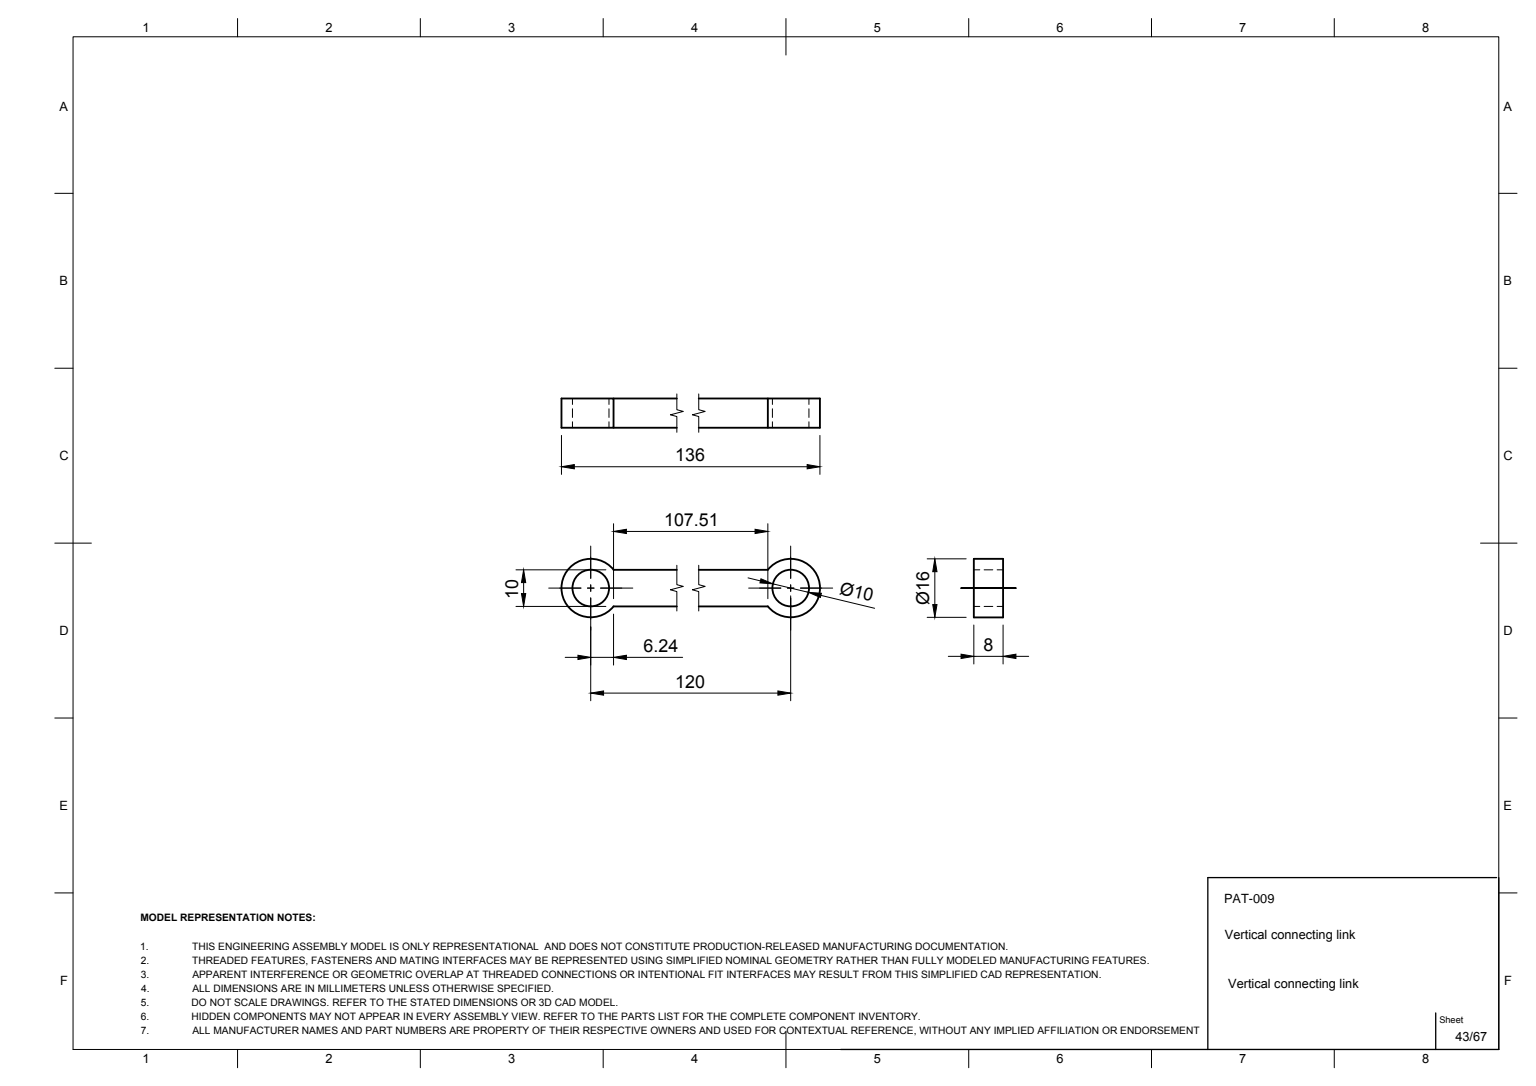
ISO-10303-21;
HEADER;
/* Generated by software containing ST-Developer
 * from STEP Tools, Inc. (www.steptools.com) 
 */

FILE_DESCRIPTION(
/* description */ ('Bell-crank linkage with push rods'),
/* implementation_level */ '2;1');

FILE_NAME(
/* name */ 'Vertical connecting link.step',
/* time_stamp */ '2026-10-28T03:25:15-07:00',
/* author */ (''),
/* organization */ (''),
/* preprocessor_version */ 'ST-DEVELOPER v20.2',
/* originating_system */ 'Autodesk Translation Framework v15.17.0.0',
/* authorisation */ '');

FILE_SCHEMA (('AUTOMOTIVE_DESIGN { 1 0 10303 214 3 1 1 }'));
ENDSEC;

DATA;
#10=MECHANICAL_DESIGN_GEOMETRIC_PRESENTATION_REPRESENTATION('',(#646),#16678);
#530=SHAPE_REPRESENTATION_RELATIONSHIP('SRR','None',#16950,#584);
#584=ADVANCED_BREP_SHAPE_REPRESENTATION('',(#706),#16655);
#646=STYLED_ITEM('',(#17277),#706);
#706=MANIFOLD_SOLID_BREP('Body1',#8838);
#866=FACE_BOUND('',#2268,.T.);
#867=FACE_BOUND('',#2269,.T.);
#868=FACE_BOUND('',#2273,.T.);
#869=FACE_BOUND('',#2274,.T.);
#1151=PLANE('',#10206);
#1152=PLANE('',#10207);
#1153=PLANE('',#10209);
#1154=PLANE('',#10212);
#1600=FACE_OUTER_BOUND('',#2263,.T.);
#1601=FACE_OUTER_BOUND('',#2264,.T.);
#1602=FACE_OUTER_BOUND('',#2265,.T.);
#1603=FACE_OUTER_BOUND('',#2266,.T.);
#1604=FACE_OUTER_BOUND('',#2267,.T.);
#1605=FACE_OUTER_BOUND('',#2270,.T.);
#1606=FACE_OUTER_BOUND('',#2271,.T.);
#1607=FACE_OUTER_BOUND('',#2272,.T.);
#2263=EDGE_LOOP('',(#7395,#7396,#7397,#7398));
#2264=EDGE_LOOP('',(#7399,#7400,#7401,#7402));
#2265=EDGE_LOOP('',(#7403,#7404,#7405,#7406));
#2266=EDGE_LOOP('',(#7407,#7408,#7409,#7410));
#2267=EDGE_LOOP('',(#7411,#7412,#7413,#7414));
#2268=EDGE_LOOP('',(#7415));
#2269=EDGE_LOOP('',(#7416));
#2270=EDGE_LOOP('',(#7417,#7418,#7419,#7420));
#2271=EDGE_LOOP('',(#7421,#7422,#7423,#7424));
#2272=EDGE_LOOP('',(#7425,#7426,#7427,#7428));
#2273=EDGE_LOOP('',(#7429));
#2274=EDGE_LOOP('',(#7430));
#2894=LINE('',#15712,#3443);
#2895=LINE('',#15718,#3444);
#2896=LINE('',#15723,#3445);
#2897=LINE('',#15727,#3446);
#2898=LINE('',#15731,#3447);
#2899=LINE('',#15733,#3448);
#2900=LINE('',#15734,#3449);
#2901=LINE('',#15737,#3450);
#2902=LINE('',#15741,#3451);
#2903=LINE('',#15742,#3452);
#3443=VECTOR('',#12482,0.5);
#3444=VECTOR('',#12489,0.5);
#3445=VECTOR('',#12494,1.);
#3446=VECTOR('',#12497,1.);
#3447=VECTOR('',#12502,1.);
#3448=VECTOR('',#12503,1.);
#3449=VECTOR('',#12504,1.);
#3450=VECTOR('',#12507,1.);
#3451=VECTOR('',#12512,1.);
#3452=VECTOR('',#12513,1.);
#3971=CIRCLE('',#10198,0.5);
#3972=CIRCLE('',#10199,0.5);
#3973=CIRCLE('',#10201,0.5);
#3974=CIRCLE('',#10202,0.5);
#3975=CIRCLE('',#10204,0.8);
#3976=CIRCLE('',#10205,0.8);
#3977=CIRCLE('',#10208,0.8);
#3978=CIRCLE('',#10211,0.8);
#4610=VERTEX_POINT('',#15709);
#4611=VERTEX_POINT('',#15711);
#4612=VERTEX_POINT('',#15715);
#4613=VERTEX_POINT('',#15717);
#4614=VERTEX_POINT('',#15721);
#4615=VERTEX_POINT('',#15722);
#4616=VERTEX_POINT('',#15724);
#4617=VERTEX_POINT('',#15726);
#4618=VERTEX_POINT('',#15730);
#4619=VERTEX_POINT('',#15732);
#4620=VERTEX_POINT('',#15736);
#4621=VERTEX_POINT('',#15740);
#5575=EDGE_CURVE('',#4610,#4610,#3971,.T.);
#5576=EDGE_CURVE('',#4610,#4611,#2894,.T.);
#5577=EDGE_CURVE('',#4611,#4611,#3972,.T.);
#5578=EDGE_CURVE('',#4612,#4612,#3973,.T.);
#5579=EDGE_CURVE('',#4612,#4613,#2895,.T.);
#5580=EDGE_CURVE('',#4613,#4613,#3974,.T.);
#5581=EDGE_CURVE('',#4614,#4615,#2896,.T.);
#5582=EDGE_CURVE('',#4616,#4614,#3975,.T.);
#5583=EDGE_CURVE('',#4617,#4616,#2897,.T.);
#5584=EDGE_CURVE('',#4617,#4615,#3976,.T.);
#5585=EDGE_CURVE('',#4618,#4615,#2898,.T.);
#5586=EDGE_CURVE('',#4619,#4618,#2899,.T.);
#5587=EDGE_CURVE('',#4614,#4619,#2900,.T.);
#5588=EDGE_CURVE('',#4617,#4620,#2901,.T.);
#5589=EDGE_CURVE('',#4618,#4620,#3977,.T.);
#5590=EDGE_CURVE('',#4621,#4616,#2902,.T.);
#5591=EDGE_CURVE('',#4620,#4621,#2903,.T.);
#5592=EDGE_CURVE('',#4619,#4621,#3978,.T.);
#7395=ORIENTED_EDGE('',*,*,#5575,.F.);
#7396=ORIENTED_EDGE('',*,*,#5576,.T.);
#7397=ORIENTED_EDGE('',*,*,#5577,.F.);
#7398=ORIENTED_EDGE('',*,*,#5576,.F.);
#7399=ORIENTED_EDGE('',*,*,#5578,.F.);
#7400=ORIENTED_EDGE('',*,*,#5579,.T.);
#7401=ORIENTED_EDGE('',*,*,#5580,.F.);
#7402=ORIENTED_EDGE('',*,*,#5579,.F.);
#7403=ORIENTED_EDGE('',*,*,#5581,.F.);
#7404=ORIENTED_EDGE('',*,*,#5582,.F.);
#7405=ORIENTED_EDGE('',*,*,#5583,.F.);
#7406=ORIENTED_EDGE('',*,*,#5584,.T.);
#7407=ORIENTED_EDGE('',*,*,#5581,.T.);
#7408=ORIENTED_EDGE('',*,*,#5585,.F.);
#7409=ORIENTED_EDGE('',*,*,#5586,.F.);
#7410=ORIENTED_EDGE('',*,*,#5587,.F.);
#7411=ORIENTED_EDGE('',*,*,#5584,.F.);
#7412=ORIENTED_EDGE('',*,*,#5588,.T.);
#7413=ORIENTED_EDGE('',*,*,#5589,.F.);
#7414=ORIENTED_EDGE('',*,*,#5585,.T.);
#7415=ORIENTED_EDGE('',*,*,#5575,.T.);
#7416=ORIENTED_EDGE('',*,*,#5578,.T.);
#7417=ORIENTED_EDGE('',*,*,#5583,.T.);
#7418=ORIENTED_EDGE('',*,*,#5590,.F.);
#7419=ORIENTED_EDGE('',*,*,#5591,.F.);
#7420=ORIENTED_EDGE('',*,*,#5588,.F.);
#7421=ORIENTED_EDGE('',*,*,#5586,.T.);
#7422=ORIENTED_EDGE('',*,*,#5589,.T.);
#7423=ORIENTED_EDGE('',*,*,#5591,.T.);
#7424=ORIENTED_EDGE('',*,*,#5592,.F.);
#7425=ORIENTED_EDGE('',*,*,#5587,.T.);
#7426=ORIENTED_EDGE('',*,*,#5592,.T.);
#7427=ORIENTED_EDGE('',*,*,#5590,.T.);
#7428=ORIENTED_EDGE('',*,*,#5582,.T.);
#7429=ORIENTED_EDGE('',*,*,#5577,.T.);
#7430=ORIENTED_EDGE('',*,*,#5580,.T.);
#8202=CYLINDRICAL_SURFACE('',#10197,0.5);
#8203=CYLINDRICAL_SURFACE('',#10200,0.5);
#8204=CYLINDRICAL_SURFACE('',#10203,0.8);
#8205=CYLINDRICAL_SURFACE('',#10210,0.8);
#8625=ADVANCED_FACE('',(#1600),#8202,.F.);
#8626=ADVANCED_FACE('',(#1601),#8203,.F.);
#8627=ADVANCED_FACE('',(#1602),#8204,.T.);
#8628=ADVANCED_FACE('',(#1603),#1151,.T.);
#8629=ADVANCED_FACE('',(#1604,#866,#867),#1152,.F.);
#8630=ADVANCED_FACE('',(#1605),#1153,.T.);
#8631=ADVANCED_FACE('',(#1606),#8205,.T.);
#8632=ADVANCED_FACE('',(#1607,#868,#869),#1154,.T.);
#8838=CLOSED_SHELL('',(#8625,#8626,#8627,#8628,#8629,#8630,#8631,#8632));
#10196=AXIS2_PLACEMENT_3D('',#15707,#12476,#12477);
#10197=AXIS2_PLACEMENT_3D('',#15708,#12478,#12479);
#10198=AXIS2_PLACEMENT_3D('',#15710,#12480,#12481);
#10199=AXIS2_PLACEMENT_3D('',#15713,#12483,#12484);
#10200=AXIS2_PLACEMENT_3D('',#15714,#12485,#12486);
#10201=AXIS2_PLACEMENT_3D('',#15716,#12487,#12488);
#10202=AXIS2_PLACEMENT_3D('',#15719,#12490,#12491);
#10203=AXIS2_PLACEMENT_3D('',#15720,#12492,#12493);
#10204=AXIS2_PLACEMENT_3D('',#15725,#12495,#12496);
#10205=AXIS2_PLACEMENT_3D('',#15728,#12498,#12499);
#10206=AXIS2_PLACEMENT_3D('',#15729,#12500,#12501);
#10207=AXIS2_PLACEMENT_3D('',#15735,#12505,#12506);
#10208=AXIS2_PLACEMENT_3D('',#15738,#12508,#12509);
#10209=AXIS2_PLACEMENT_3D('',#15739,#12510,#12511);
#10210=AXIS2_PLACEMENT_3D('',#15743,#12514,#12515);
#10211=AXIS2_PLACEMENT_3D('',#15744,#12516,#12517);
#10212=AXIS2_PLACEMENT_3D('',#15745,#12518,#12519);
#12476=DIRECTION('axis',(0.,0.,1.));
#12477=DIRECTION('refdir',(1.,0.,0.));
#12478=DIRECTION('center_axis',(0.,0.,1.));
#12479=DIRECTION('ref_axis',(1.,0.,0.));
#12480=DIRECTION('center_axis',(0.,0.,1.));
#12481=DIRECTION('ref_axis',(1.,0.,0.));
#12482=DIRECTION('',(0.,0.,1.));
#12483=DIRECTION('center_axis',(0.,0.,-1.));
#12484=DIRECTION('ref_axis',(1.,0.,0.));
#12485=DIRECTION('center_axis',(0.,0.,1.));
#12486=DIRECTION('ref_axis',(1.,0.,0.));
#12487=DIRECTION('center_axis',(0.,0.,1.));
#12488=DIRECTION('ref_axis',(1.,0.,0.));
#12489=DIRECTION('',(0.,0.,1.));
#12490=DIRECTION('center_axis',(0.,0.,-1.));
#12491=DIRECTION('ref_axis',(1.,0.,0.));
#12492=DIRECTION('center_axis',(0.,0.,1.));
#12493=DIRECTION('ref_axis',(-1.83697019872103E-16,1.,0.));
#12494=DIRECTION('',(0.,0.,-1.));
#12495=DIRECTION('center_axis',(0.,0.,1.));
#12496=DIRECTION('ref_axis',(1.,0.,0.));
#12497=DIRECTION('',(0.,0.,1.));
#12498=DIRECTION('center_axis',(0.,0.,1.));
#12499=DIRECTION('ref_axis',(1.,0.,0.));
#12500=DIRECTION('center_axis',(-1.,0.,0.));
#12501=DIRECTION('ref_axis',(0.,-1.,0.));
#12502=DIRECTION('',(0.,1.,0.));
#12503=DIRECTION('',(0.,0.,-1.));
#12504=DIRECTION('',(0.,-1.,0.));
#12505=DIRECTION('center_axis',(0.,0.,1.));
#12506=DIRECTION('ref_axis',(1.,0.,0.));
#12507=DIRECTION('',(0.,-1.,0.));
#12508=DIRECTION('center_axis',(0.,0.,1.));
#12509=DIRECTION('ref_axis',(1.,0.,0.));
#12510=DIRECTION('center_axis',(1.,0.,0.));
#12511=DIRECTION('ref_axis',(0.,1.,0.));
#12512=DIRECTION('',(0.,1.,0.));
#12513=DIRECTION('',(0.,0.,1.));
#12514=DIRECTION('center_axis',(0.,0.,1.));
#12515=DIRECTION('ref_axis',(-1.83697019872103E-16,-1.,0.));
#12516=DIRECTION('center_axis',(0.,0.,1.));
#12517=DIRECTION('ref_axis',(1.,0.,0.));
#12518=DIRECTION('center_axis',(0.,0.,1.));
#12519=DIRECTION('ref_axis',(1.,0.,0.));
#15707=CARTESIAN_POINT('',(0.,0.,0.));
#15708=CARTESIAN_POINT('Origin',(4.,0.,6.7));
#15709=CARTESIAN_POINT('',(3.5,-6.12323399573677E-17,6.8));
#15710=CARTESIAN_POINT('Origin',(4.,0.,6.8));
#15711=CARTESIAN_POINT('',(3.5,6.12323399573677E-17,7.6));
#15712=CARTESIAN_POINT('',(3.5,-6.12323399573677E-17,6.7));
#15713=CARTESIAN_POINT('Origin',(4.,0.,7.6));
#15714=CARTESIAN_POINT('Origin',(4.,12.,6.7));
#15715=CARTESIAN_POINT('',(3.5,12.,6.8));
#15716=CARTESIAN_POINT('Origin',(4.,12.,6.8));
#15717=CARTESIAN_POINT('',(3.5,12.,7.6));
#15718=CARTESIAN_POINT('',(3.5,12.,6.7));
#15719=CARTESIAN_POINT('Origin',(4.,12.,7.6));
#15720=CARTESIAN_POINT('Origin',(4.,12.,6.8));
#15721=CARTESIAN_POINT('',(3.5,11.3755002001602,7.6));
#15722=CARTESIAN_POINT('',(3.5,11.3755002001602,6.8));
#15723=CARTESIAN_POINT('',(3.5,11.3755002001602,6.8));
#15724=CARTESIAN_POINT('',(4.5,11.3755002001602,7.6));
#15725=CARTESIAN_POINT('Origin',(4.,12.,7.6));
#15726=CARTESIAN_POINT('',(4.5,11.3755002001602,6.8));
#15727=CARTESIAN_POINT('',(4.5,11.3755002001602,6.8));
#15728=CARTESIAN_POINT('Origin',(4.,12.,6.8));
#15729=CARTESIAN_POINT('Origin',(3.5,12.,6.8));
#15730=CARTESIAN_POINT('',(3.5,0.62449979983984,6.8));
#15731=CARTESIAN_POINT('',(3.5,0.,6.8));
#15732=CARTESIAN_POINT('',(3.5,0.62449979983984,7.6));
#15733=CARTESIAN_POINT('',(3.5,0.62449979983984,6.8));
#15734=CARTESIAN_POINT('',(3.5,0.,7.6));
#15735=CARTESIAN_POINT('Origin',(4.,0.,6.8));
#15736=CARTESIAN_POINT('',(4.5,0.62449979983984,6.8));
#15737=CARTESIAN_POINT('',(4.5,12.,6.8));
#15738=CARTESIAN_POINT('Origin',(4.,0.,6.8));
#15739=CARTESIAN_POINT('Origin',(4.5,0.,6.8));
#15740=CARTESIAN_POINT('',(4.5,0.62449979983984,7.6));
#15741=CARTESIAN_POINT('',(4.5,12.,7.6));
#15742=CARTESIAN_POINT('',(4.5,0.62449979983984,6.8));
#15743=CARTESIAN_POINT('Origin',(4.,0.,6.8));
#15744=CARTESIAN_POINT('Origin',(4.,0.,7.6));
#15745=CARTESIAN_POINT('Origin',(4.,0.,7.6));
#16591=UNCERTAINTY_MEASURE_WITH_UNIT(LENGTH_MEASURE(0.001),#16679,
'DISTANCE_ACCURACY_VALUE',
'Maximum model space distance between geometric entities at asserted c
onnectivities');
#16614=UNCERTAINTY_MEASURE_WITH_UNIT(LENGTH_MEASURE(0.001),#16679,
'DISTANCE_ACCURACY_VALUE',
'Maximum model space distance between geometric entities at asserted c
onnectivities');
#16655=(
GEOMETRIC_REPRESENTATION_CONTEXT(3)
GLOBAL_UNCERTAINTY_ASSIGNED_CONTEXT((#16591))
GLOBAL_UNIT_ASSIGNED_CONTEXT((#16679,#16681,#16682))
REPRESENTATION_CONTEXT('','3D')
);
#16678=(
GEOMETRIC_REPRESENTATION_CONTEXT(3)
GLOBAL_UNCERTAINTY_ASSIGNED_CONTEXT((#16614))
GLOBAL_UNIT_ASSIGNED_CONTEXT((#16679,#16681,#16682))
REPRESENTATION_CONTEXT('','3D')
);
#16679=(
LENGTH_UNIT()
NAMED_UNIT(*)
SI_UNIT(.CENTI.,.METRE.)
);
#16681=(
NAMED_UNIT(*)
PLANE_ANGLE_UNIT()
SI_UNIT($,.RADIAN.)
);
#16682=(
NAMED_UNIT(*)
SI_UNIT($,.STERADIAN.)
SOLID_ANGLE_UNIT()
);
#16723=SHAPE_DEFINITION_REPRESENTATION(#16794,#16950);
#16794=PRODUCT_DEFINITION_SHAPE('',$,#17014);
#16950=SHAPE_REPRESENTATION('',(#10196),#16655);
#16973=PRODUCT_DEFINITION_CONTEXT('part definition',#17164,'design');
#17014=PRODUCT_DEFINITION('Vertical connecting link',
'Vertical connecting link',#17077,#16973);
#17077=PRODUCT_DEFINITION_FORMATION('',$,#17206);
#17164=APPLICATION_CONTEXT(
'Core Data for Automotive Mechanical Design Process');
#17165=PRODUCT_CONTEXT('part definition',#17164,'mechanical');
#17206=PRODUCT('Vertical connecting link','Vertical connecting link',
'Vertical connecting link',(#17165));
#17271=COLOUR_RGB('Light Blue',0.38,0.62,0.78);
#17272=FILL_AREA_STYLE_COLOUR('',#17271);
#17273=FILL_AREA_STYLE('',(#17272));
#17274=SURFACE_STYLE_FILL_AREA(#17273);
#17275=SURFACE_SIDE_STYLE('',(#17274));
#17276=SURFACE_STYLE_USAGE(.BOTH.,#17275);
#17277=PRESENTATION_STYLE_ASSIGNMENT((#17276));
ENDSEC;
END-ISO-10303-21;
